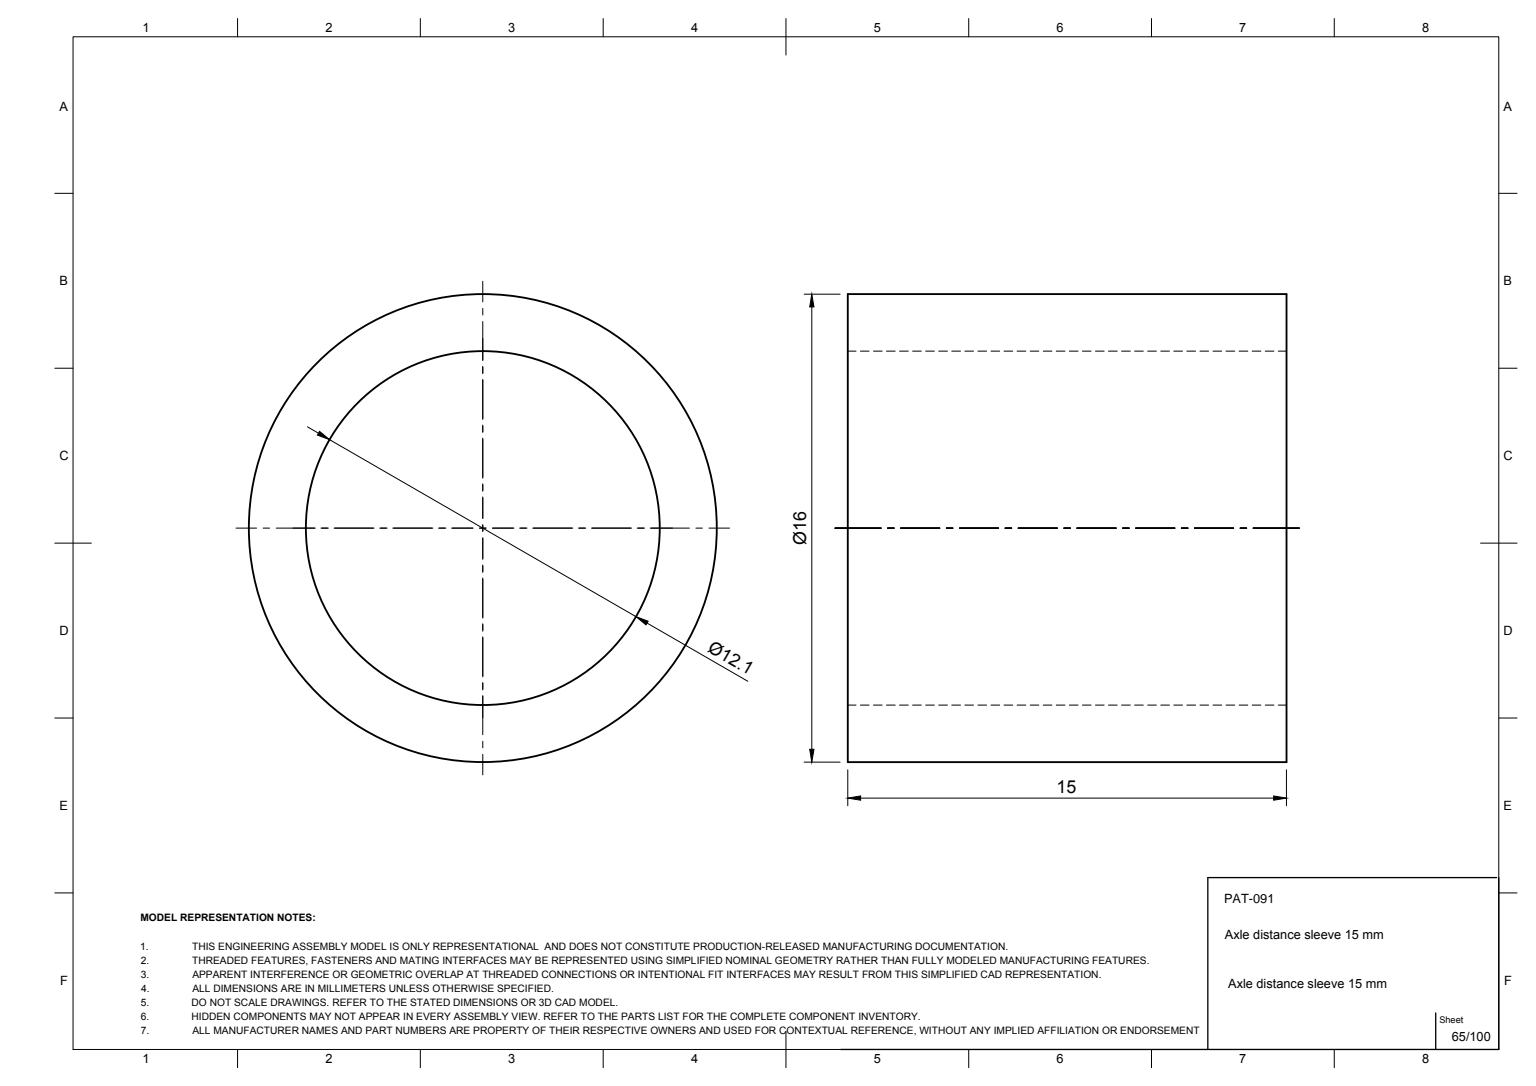
ISO-10303-21;
HEADER;
/* Generated by software containing ST-Developer
 * from STEP Tools, Inc. (www.steptools.com) 
 */

FILE_DESCRIPTION(
/* description */ ('PAT-091'),
/* implementation_level */ '2;1');

FILE_NAME(
/* name */ 'Axle distance sleeve 15 mm.step',
/* time_stamp */ '2026-10-27T15:34:44-07:00',
/* author */ (''),
/* organization */ (''),
/* preprocessor_version */ 'ST-DEVELOPER v20.2',
/* originating_system */ 'Autodesk Translation Framework v15.17.0.0',
/* authorisation */ '');

FILE_SCHEMA (('AUTOMOTIVE_DESIGN { 1 0 10303 214 3 1 1 }'));
ENDSEC;

DATA;
#10=MECHANICAL_DESIGN_GEOMETRIC_PRESENTATION_REPRESENTATION('',(#1022),#25100);
#802=SHAPE_REPRESENTATION_RELATIONSHIP('SRR','None',#25566,#912);
#912=ADVANCED_BREP_SHAPE_REPRESENTATION('',(#1144),#25036);
#1022=STYLED_ITEM('',(#26191),#1144);
#1144=MANIFOLD_SOLID_BREP('Body1',#13301);
#1468=FACE_BOUND('',#3541,.T.);
#1469=FACE_BOUND('',#3543,.T.);
#1865=PLANE('',#15407);
#1866=PLANE('',#15408);
#2467=FACE_OUTER_BOUND('',#3538,.T.);
#2468=FACE_OUTER_BOUND('',#3539,.T.);
#2469=FACE_OUTER_BOUND('',#3540,.T.);
#2470=FACE_OUTER_BOUND('',#3542,.T.);
#3538=EDGE_LOOP('',(#10608,#10609,#10610,#10611));
#3539=EDGE_LOOP('',(#10612,#10613,#10614,#10615));
#3540=EDGE_LOOP('',(#10616));
#3541=EDGE_LOOP('',(#10617));
#3542=EDGE_LOOP('',(#10618));
#3543=EDGE_LOOP('',(#10619));
#4583=LINE('',#22852,#5323);
#4584=LINE('',#22858,#5324);
#5323=VECTOR('',#18563,0.604999999999997);
#5324=VECTOR('',#18570,0.799999999999997);
#5959=CIRCLE('',#15402,0.604999999999997);
#5960=CIRCLE('',#15403,0.604999999999997);
#5961=CIRCLE('',#15405,0.799999999999997);
#5962=CIRCLE('',#15406,0.799999999999997);
#6926=VERTEX_POINT('',#22849);
#6927=VERTEX_POINT('',#22851);
#6928=VERTEX_POINT('',#22855);
#6929=VERTEX_POINT('',#22857);
#8239=EDGE_CURVE('',#6926,#6926,#5959,.T.);
#8240=EDGE_CURVE('',#6926,#6927,#4583,.T.);
#8241=EDGE_CURVE('',#6927,#6927,#5960,.T.);
#8242=EDGE_CURVE('',#6928,#6928,#5961,.T.);
#8243=EDGE_CURVE('',#6928,#6929,#4584,.T.);
#8244=EDGE_CURVE('',#6929,#6929,#5962,.T.);
#10608=ORIENTED_EDGE('',*,*,#8239,.F.);
#10609=ORIENTED_EDGE('',*,*,#8240,.T.);
#10610=ORIENTED_EDGE('',*,*,#8241,.T.);
#10611=ORIENTED_EDGE('',*,*,#8240,.F.);
#10612=ORIENTED_EDGE('',*,*,#8242,.F.);
#10613=ORIENTED_EDGE('',*,*,#8243,.T.);
#10614=ORIENTED_EDGE('',*,*,#8244,.T.);
#10615=ORIENTED_EDGE('',*,*,#8243,.F.);
#10616=ORIENTED_EDGE('',*,*,#8242,.T.);
#10617=ORIENTED_EDGE('',*,*,#8239,.T.);
#10618=ORIENTED_EDGE('',*,*,#8244,.F.);
#10619=ORIENTED_EDGE('',*,*,#8241,.F.);
#12246=CYLINDRICAL_SURFACE('',#15401,0.604999999999997);
#12247=CYLINDRICAL_SURFACE('',#15404,0.799999999999997);
#12834=ADVANCED_FACE('',(#2467),#12246,.F.);
#12835=ADVANCED_FACE('',(#2468),#12247,.T.);
#12836=ADVANCED_FACE('',(#2469,#1468),#1865,.T.);
#12837=ADVANCED_FACE('',(#2470,#1469),#1866,.F.);
#13301=CLOSED_SHELL('',(#12834,#12835,#12836,#12837));
#15400=AXIS2_PLACEMENT_3D('',#22847,#18557,#18558);
#15401=AXIS2_PLACEMENT_3D('',#22848,#18559,#18560);
#15402=AXIS2_PLACEMENT_3D('',#22850,#18561,#18562);
#15403=AXIS2_PLACEMENT_3D('',#22853,#18564,#18565);
#15404=AXIS2_PLACEMENT_3D('',#22854,#18566,#18567);
#15405=AXIS2_PLACEMENT_3D('',#22856,#18568,#18569);
#15406=AXIS2_PLACEMENT_3D('',#22859,#18571,#18572);
#15407=AXIS2_PLACEMENT_3D('',#22860,#18573,#18574);
#15408=AXIS2_PLACEMENT_3D('',#22861,#18575,#18576);
#18557=DIRECTION('axis',(0.,0.,1.));
#18558=DIRECTION('refdir',(1.,0.,0.));
#18559=DIRECTION('center_axis',(0.,1.,0.));
#18560=DIRECTION('ref_axis',(1.,0.,0.));
#18561=DIRECTION('center_axis',(0.,-1.,0.));
#18562=DIRECTION('ref_axis',(1.,0.,0.));
#18563=DIRECTION('',(0.,-1.,0.));
#18564=DIRECTION('center_axis',(0.,-1.,0.));
#18565=DIRECTION('ref_axis',(1.,0.,0.));
#18566=DIRECTION('center_axis',(0.,1.,0.));
#18567=DIRECTION('ref_axis',(1.,0.,0.));
#18568=DIRECTION('center_axis',(0.,1.,0.));
#18569=DIRECTION('ref_axis',(1.,0.,0.));
#18570=DIRECTION('',(0.,-1.,0.));
#18571=DIRECTION('center_axis',(0.,1.,0.));
#18572=DIRECTION('ref_axis',(1.,0.,0.));
#18573=DIRECTION('center_axis',(0.,1.,0.));
#18574=DIRECTION('ref_axis',(1.,0.,0.));
#18575=DIRECTION('center_axis',(0.,1.,0.));
#18576=DIRECTION('ref_axis',(1.,0.,0.));
#22847=CARTESIAN_POINT('',(0.,0.,0.));
#22848=CARTESIAN_POINT('Origin',(38.7298334620742,3.5,13.));
#22849=CARTESIAN_POINT('',(38.1248334620742,5.,13.));
#22850=CARTESIAN_POINT('Origin',(38.7298334620742,5.,13.));
#22851=CARTESIAN_POINT('',(38.1248334620742,3.5,13.));
#22852=CARTESIAN_POINT('',(38.1248334620742,3.5,13.));
#22853=CARTESIAN_POINT('Origin',(38.7298334620742,3.5,13.));
#22854=CARTESIAN_POINT('Origin',(38.7298334620742,3.5,13.));
#22855=CARTESIAN_POINT('',(37.9298334620742,5.,13.));
#22856=CARTESIAN_POINT('Origin',(38.7298334620742,5.,13.));
#22857=CARTESIAN_POINT('',(37.9298334620742,3.5,13.));
#22858=CARTESIAN_POINT('',(37.9298334620742,3.5,13.));
#22859=CARTESIAN_POINT('Origin',(38.7298334620742,3.5,13.));
#22860=CARTESIAN_POINT('Origin',(38.7298334620742,5.,13.));
#22861=CARTESIAN_POINT('Origin',(38.7298334620742,3.5,13.));
#24915=UNCERTAINTY_MEASURE_WITH_UNIT(LENGTH_MEASURE(0.001),#25101,
'DISTANCE_ACCURACY_VALUE',
'Maximum model space distance between geometric entities at asserted c
onnectivities');
#24979=UNCERTAINTY_MEASURE_WITH_UNIT(LENGTH_MEASURE(0.001),#25101,
'DISTANCE_ACCURACY_VALUE',
'Maximum model space distance between geometric entities at asserted c
onnectivities');
#25036=(
GEOMETRIC_REPRESENTATION_CONTEXT(3)
GLOBAL_UNCERTAINTY_ASSIGNED_CONTEXT((#24915))
GLOBAL_UNIT_ASSIGNED_CONTEXT((#25101,#25103,#25104))
REPRESENTATION_CONTEXT('','3D')
);
#25100=(
GEOMETRIC_REPRESENTATION_CONTEXT(3)
GLOBAL_UNCERTAINTY_ASSIGNED_CONTEXT((#24979))
GLOBAL_UNIT_ASSIGNED_CONTEXT((#25101,#25103,#25104))
REPRESENTATION_CONTEXT('','3D')
);
#25101=(
LENGTH_UNIT()
NAMED_UNIT(*)
SI_UNIT(.CENTI.,.METRE.)
);
#25103=(
NAMED_UNIT(*)
PLANE_ANGLE_UNIT()
SI_UNIT($,.RADIAN.)
);
#25104=(
NAMED_UNIT(*)
SI_UNIT($,.STERADIAN.)
SOLID_ANGLE_UNIT()
);
#25161=SHAPE_DEFINITION_REPRESENTATION(#25281,#25566);
#25281=PRODUCT_DEFINITION_SHAPE('',$,#25687);
#25566=SHAPE_REPRESENTATION('',(#15400),#25036);
#25630=PRODUCT_DEFINITION_CONTEXT('part definition',#25992,'design');
#25687=PRODUCT_DEFINITION('Axle distance sleeve 15 mm',
'Axle distance sleeve 15 mm',#25807,#25630);
#25807=PRODUCT_DEFINITION_FORMATION('',$,#26050);
#25992=APPLICATION_CONTEXT(
'Core Data for Automotive Mechanical Design Process');
#25993=PRODUCT_CONTEXT('part definition',#25992,'mechanical');
#26050=PRODUCT('Axle distance sleeve 15 mm',
'Axle distance sleeve 15 mm','Axle distance sleeve 15 mm',(#25993));
#26185=COLOUR_RGB('Grey',0.48,0.52,0.57);
#26186=FILL_AREA_STYLE_COLOUR('',#26185);
#26187=FILL_AREA_STYLE('',(#26186));
#26188=SURFACE_STYLE_FILL_AREA(#26187);
#26189=SURFACE_SIDE_STYLE('',(#26188));
#26190=SURFACE_STYLE_USAGE(.BOTH.,#26189);
#26191=PRESENTATION_STYLE_ASSIGNMENT((#26190));
ENDSEC;
END-ISO-10303-21;
